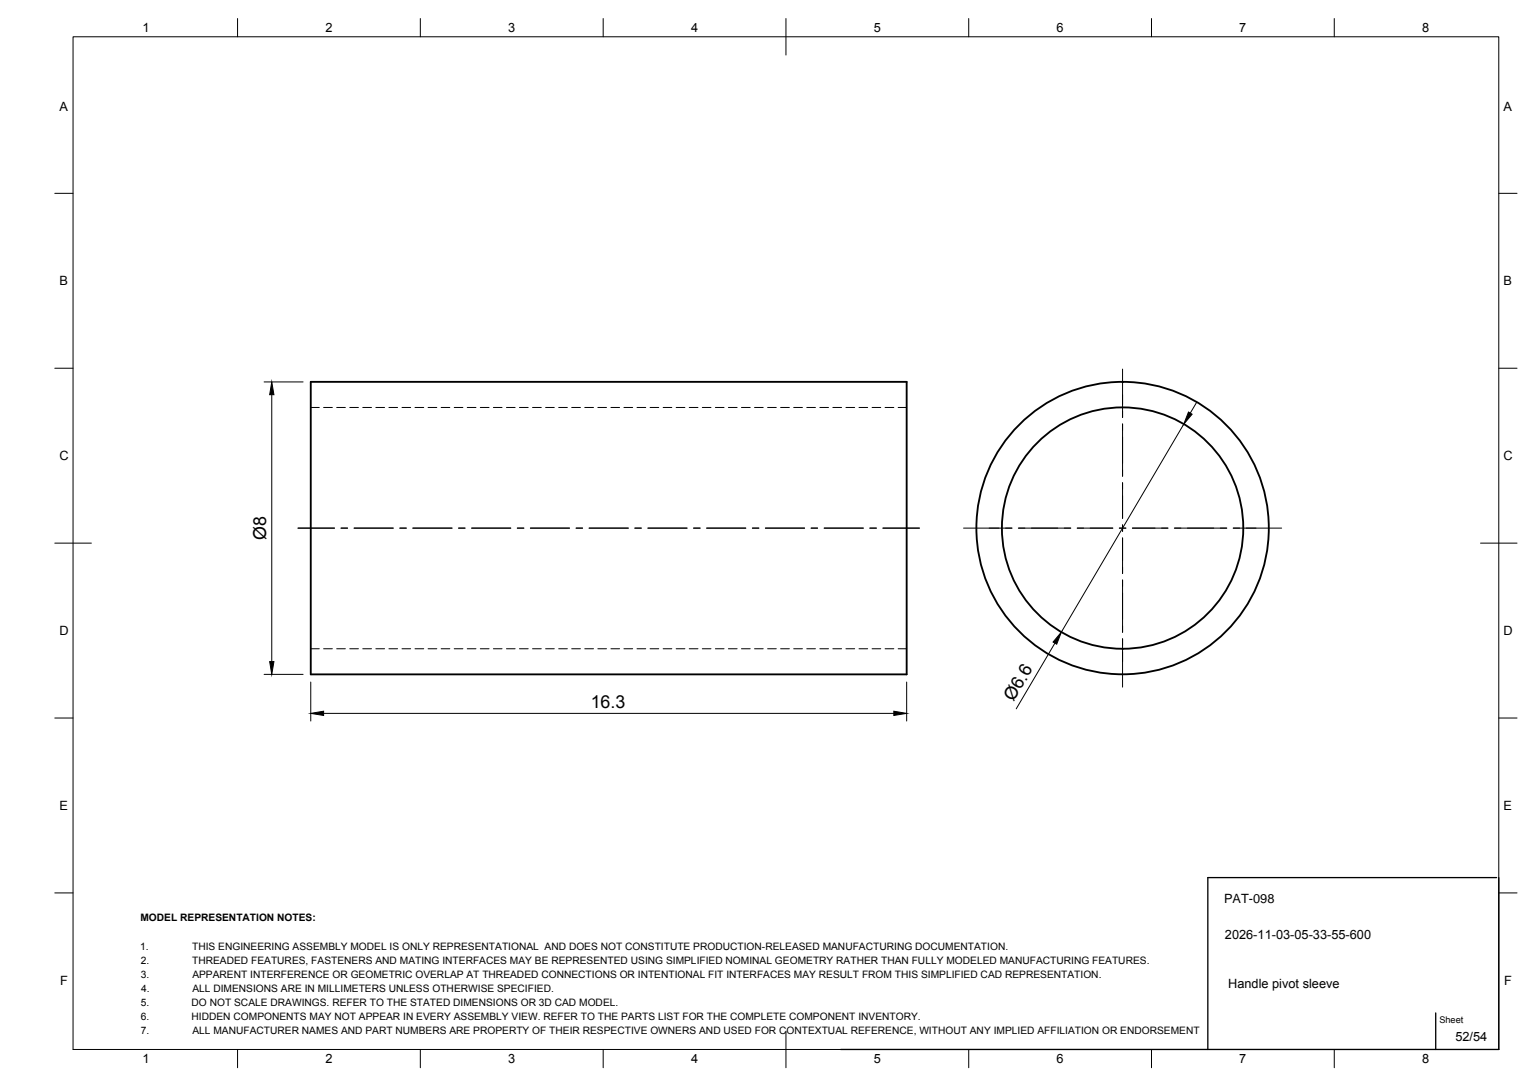
ISO-10303-21;
HEADER;
/* Generated by software containing ST-Developer
 * from STEP Tools, Inc. (www.steptools.com) 
 */

FILE_DESCRIPTION(
/* description */ ('Spring compression tester'),
/* implementation_level */ '2;1');

FILE_NAME(
/* name */ 'Handle pivot sleeve.step',
/* time_stamp */ '2026-10-28T03:24:11-07:00',
/* author */ (''),
/* organization */ (''),
/* preprocessor_version */ 'ST-DEVELOPER v20.2',
/* originating_system */ 'Autodesk Translation Framework v15.17.0.0',
/* authorisation */ '');

FILE_SCHEMA (('AUTOMOTIVE_DESIGN { 1 0 10303 214 3 1 1 }'));
ENDSEC;

DATA;
#10=MECHANICAL_DESIGN_GEOMETRIC_PRESENTATION_REPRESENTATION('',(#1173),#43521);
#1038=SHAPE_REPRESENTATION_RELATIONSHIP('SRR','None',#43855,#1098);
#1098=ADVANCED_BREP_SHAPE_REPRESENTATION('',(#1242),#43515);
#1173=STYLED_ITEM('',(#44195),#1242);
#1242=MANIFOLD_SOLID_BREP('Body1',#18616);
#1581=FACE_BOUND('',#4550,.T.);
#1582=FACE_BOUND('',#4552,.T.);
#2134=PLANE('',#21108);
#2135=PLANE('',#21109);
#3166=FACE_OUTER_BOUND('',#4547,.T.);
#3167=FACE_OUTER_BOUND('',#4548,.T.);
#3168=FACE_OUTER_BOUND('',#4549,.T.);
#3169=FACE_OUTER_BOUND('',#4551,.T.);
#4547=EDGE_LOOP('',(#16907,#16908,#16909,#16910));
#4548=EDGE_LOOP('',(#16911,#16912,#16913,#16914));
#4549=EDGE_LOOP('',(#16915));
#4550=EDGE_LOOP('',(#16916));
#4551=EDGE_LOOP('',(#16917));
#4552=EDGE_LOOP('',(#16918));
#5963=LINE('',#43157,#7395);
#5964=LINE('',#43163,#7396);
#7395=VECTOR('',#26193,0.33);
#7396=VECTOR('',#26200,0.4);
#8112=CIRCLE('',#21103,0.33);
#8113=CIRCLE('',#21104,0.33);
#8114=CIRCLE('',#21106,0.4);
#8115=CIRCLE('',#21107,0.4);
#9709=VERTEX_POINT('',#43154);
#9710=VERTEX_POINT('',#43156);
#9711=VERTEX_POINT('',#43160);
#9712=VERTEX_POINT('',#43162);
#12118=EDGE_CURVE('',#9709,#9709,#8112,.T.);
#12119=EDGE_CURVE('',#9709,#9710,#5963,.T.);
#12120=EDGE_CURVE('',#9710,#9710,#8113,.T.);
#12121=EDGE_CURVE('',#9711,#9711,#8114,.T.);
#12122=EDGE_CURVE('',#9711,#9712,#5964,.T.);
#12123=EDGE_CURVE('',#9712,#9712,#8115,.T.);
#16907=ORIENTED_EDGE('',*,*,#12118,.F.);
#16908=ORIENTED_EDGE('',*,*,#12119,.T.);
#16909=ORIENTED_EDGE('',*,*,#12120,.T.);
#16910=ORIENTED_EDGE('',*,*,#12119,.F.);
#16911=ORIENTED_EDGE('',*,*,#12121,.F.);
#16912=ORIENTED_EDGE('',*,*,#12122,.T.);
#16913=ORIENTED_EDGE('',*,*,#12123,.T.);
#16914=ORIENTED_EDGE('',*,*,#12122,.F.);
#16915=ORIENTED_EDGE('',*,*,#12121,.T.);
#16916=ORIENTED_EDGE('',*,*,#12118,.T.);
#16917=ORIENTED_EDGE('',*,*,#12123,.F.);
#16918=ORIENTED_EDGE('',*,*,#12120,.F.);
#17485=CYLINDRICAL_SURFACE('',#21102,0.33);
#17486=CYLINDRICAL_SURFACE('',#21105,0.4);
#18490=ADVANCED_FACE('',(#3166),#17485,.F.);
#18491=ADVANCED_FACE('',(#3167),#17486,.T.);
#18492=ADVANCED_FACE('',(#3168,#1581),#2134,.T.);
#18493=ADVANCED_FACE('',(#3169,#1582),#2135,.F.);
#18616=CLOSED_SHELL('',(#18490,#18491,#18492,#18493));
#21101=AXIS2_PLACEMENT_3D('',#43152,#26187,#26188);
#21102=AXIS2_PLACEMENT_3D('',#43153,#26189,#26190);
#21103=AXIS2_PLACEMENT_3D('',#43155,#26191,#26192);
#21104=AXIS2_PLACEMENT_3D('',#43158,#26194,#26195);
#21105=AXIS2_PLACEMENT_3D('',#43159,#26196,#26197);
#21106=AXIS2_PLACEMENT_3D('',#43161,#26198,#26199);
#21107=AXIS2_PLACEMENT_3D('',#43164,#26201,#26202);
#21108=AXIS2_PLACEMENT_3D('',#43165,#26203,#26204);
#21109=AXIS2_PLACEMENT_3D('',#43166,#26205,#26206);
#26187=DIRECTION('axis',(0.,0.,1.));
#26188=DIRECTION('refdir',(1.,0.,0.));
#26189=DIRECTION('center_axis',(1.,0.,0.));
#26190=DIRECTION('ref_axis',(0.,0.,-1.));
#26191=DIRECTION('center_axis',(-1.,0.,0.));
#26192=DIRECTION('ref_axis',(0.,0.,-1.));
#26193=DIRECTION('',(-1.,0.,0.));
#26194=DIRECTION('center_axis',(-1.,0.,0.));
#26195=DIRECTION('ref_axis',(0.,0.,-1.));
#26196=DIRECTION('center_axis',(1.,0.,0.));
#26197=DIRECTION('ref_axis',(0.,0.,-1.));
#26198=DIRECTION('center_axis',(1.,0.,0.));
#26199=DIRECTION('ref_axis',(0.,0.,-1.));
#26200=DIRECTION('',(-1.,0.,0.));
#26201=DIRECTION('center_axis',(1.,0.,0.));
#26202=DIRECTION('ref_axis',(0.,0.,-1.));
#26203=DIRECTION('center_axis',(1.,0.,0.));
#26204=DIRECTION('ref_axis',(0.,0.,-1.));
#26205=DIRECTION('center_axis',(1.,0.,0.));
#26206=DIRECTION('ref_axis',(0.,0.,-1.));
#43152=CARTESIAN_POINT('',(0.,0.,0.));
#43153=CARTESIAN_POINT('Origin',(29.4,0.,6.5));
#43154=CARTESIAN_POINT('',(31.03,-4.04133443718627E-17,6.83));
#43155=CARTESIAN_POINT('Origin',(31.03,0.,6.5));
#43156=CARTESIAN_POINT('',(29.4,-4.04133443718627E-17,6.83));
#43157=CARTESIAN_POINT('',(29.4,-4.04133443718627E-17,6.83));
#43158=CARTESIAN_POINT('Origin',(29.4,0.,6.5));
#43159=CARTESIAN_POINT('Origin',(29.4,0.,6.5));
#43160=CARTESIAN_POINT('',(31.03,-4.89858719658942E-17,6.9));
#43161=CARTESIAN_POINT('Origin',(31.03,0.,6.5));
#43162=CARTESIAN_POINT('',(29.4,-4.89858719658942E-17,6.9));
#43163=CARTESIAN_POINT('',(29.4,-4.89858719658942E-17,6.9));
#43164=CARTESIAN_POINT('Origin',(29.4,0.,6.5));
#43165=CARTESIAN_POINT('Origin',(31.03,0.,6.5));
#43166=CARTESIAN_POINT('Origin',(29.4,0.,6.5));
#43447=UNCERTAINTY_MEASURE_WITH_UNIT(LENGTH_MEASURE(0.001),#43522,
'DISTANCE_ACCURACY_VALUE',
'Maximum model space distance between geometric entities at asserted c
onnectivities');
#43453=UNCERTAINTY_MEASURE_WITH_UNIT(LENGTH_MEASURE(0.001),#43522,
'DISTANCE_ACCURACY_VALUE',
'Maximum model space distance between geometric entities at asserted c
onnectivities');
#43515=(
GEOMETRIC_REPRESENTATION_CONTEXT(3)
GLOBAL_UNCERTAINTY_ASSIGNED_CONTEXT((#43447))
GLOBAL_UNIT_ASSIGNED_CONTEXT((#43522,#43524,#43525))
REPRESENTATION_CONTEXT('','3D')
);
#43521=(
GEOMETRIC_REPRESENTATION_CONTEXT(3)
GLOBAL_UNCERTAINTY_ASSIGNED_CONTEXT((#43453))
GLOBAL_UNIT_ASSIGNED_CONTEXT((#43522,#43524,#43525))
REPRESENTATION_CONTEXT('','3D')
);
#43522=(
LENGTH_UNIT()
NAMED_UNIT(*)
SI_UNIT(.CENTI.,.METRE.)
);
#43524=(
NAMED_UNIT(*)
PLANE_ANGLE_UNIT()
SI_UNIT($,.RADIAN.)
);
#43525=(
NAMED_UNIT(*)
SI_UNIT($,.STERADIAN.)
SOLID_ANGLE_UNIT()
);
#43587=SHAPE_DEFINITION_REPRESENTATION(#43774,#43855);
#43774=PRODUCT_DEFINITION_SHAPE('',$,#43923);
#43855=SHAPE_REPRESENTATION('',(#21101),#43515);
#43861=PRODUCT_DEFINITION_CONTEXT('part definition',#44064,'design');
#43923=PRODUCT_DEFINITION('Handle pivot sleeve','Handle pivot sleeve',#43990,
#43861);
#43990=PRODUCT_DEFINITION_FORMATION('',$,#44127);
#44064=APPLICATION_CONTEXT(
'Core Data for Automotive Mechanical Design Process');
#44065=PRODUCT_CONTEXT('part definition',#44064,'mechanical');
#44127=PRODUCT('Handle pivot sleeve','Handle pivot sleeve',
'Handle pivot sleeve',(#44065));
#44189=COLOUR_RGB('Sky Blue',0.24,0.69,0.87);
#44190=FILL_AREA_STYLE_COLOUR('',#44189);
#44191=FILL_AREA_STYLE('',(#44190));
#44192=SURFACE_STYLE_FILL_AREA(#44191);
#44193=SURFACE_SIDE_STYLE('',(#44192));
#44194=SURFACE_STYLE_USAGE(.BOTH.,#44193);
#44195=PRESENTATION_STYLE_ASSIGNMENT((#44194));
ENDSEC;
END-ISO-10303-21;
